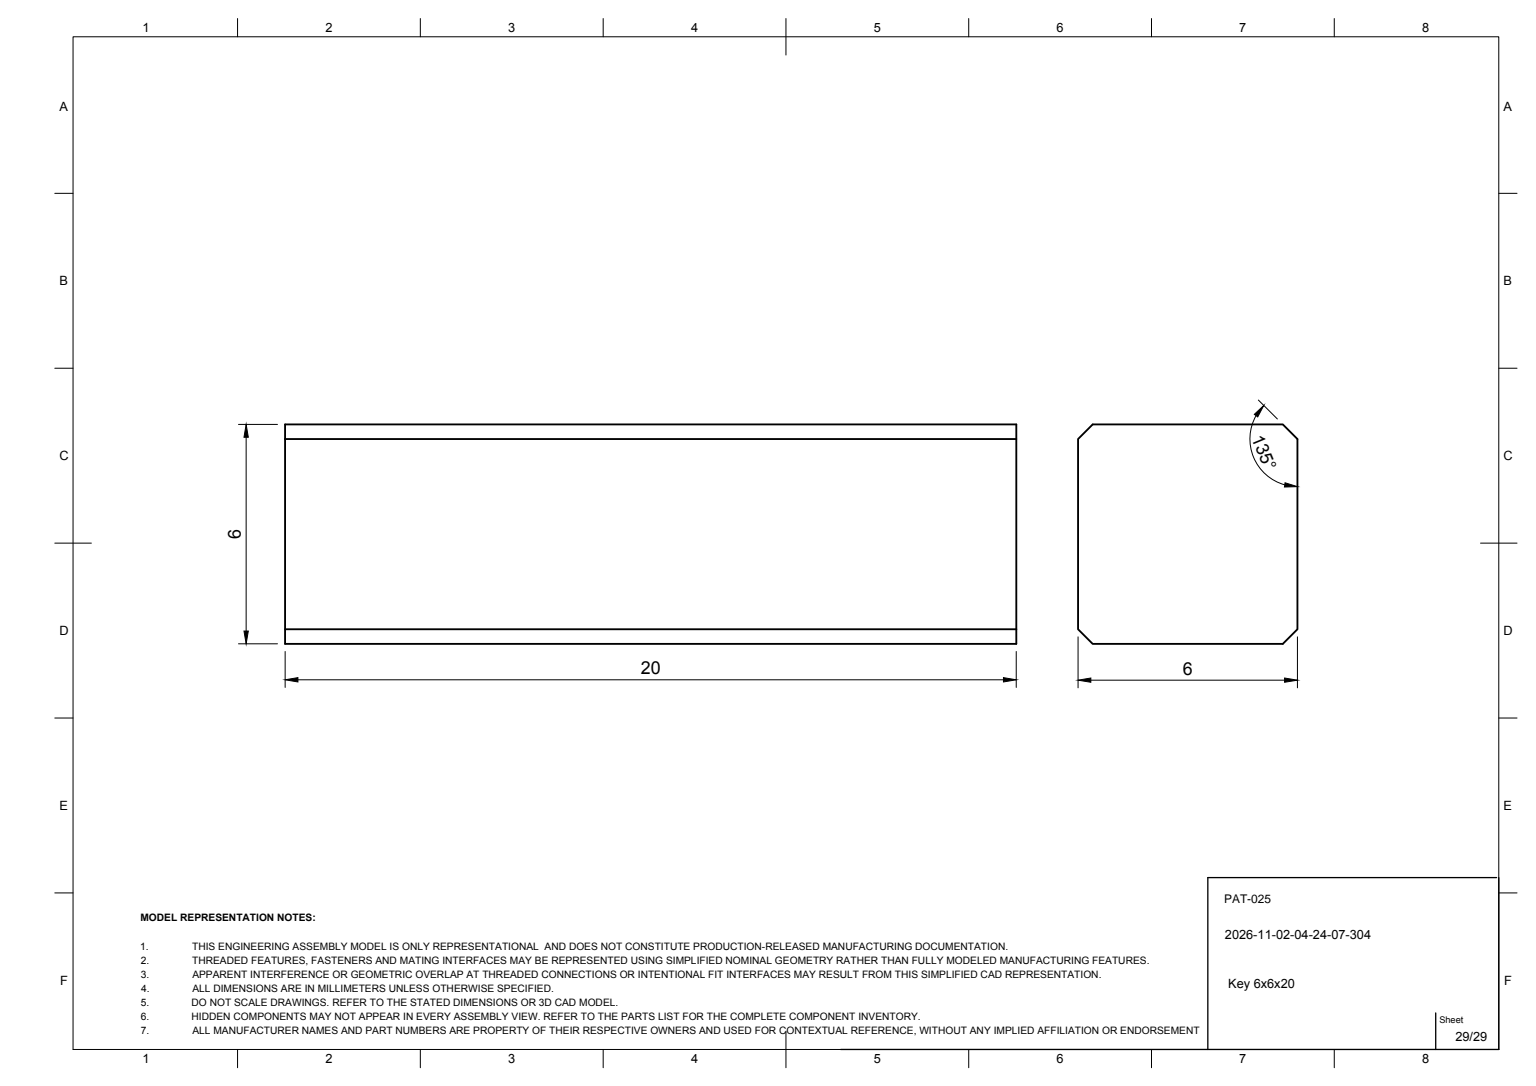
ISO-10303-21;
HEADER;
/* Generated by software containing ST-Developer
 * from STEP Tools, Inc. (www.steptools.com) 
 */

FILE_DESCRIPTION(
/* description */ ('Counter shaft with two pulleys and keyed hub'),
/* implementation_level */ '2;1');

FILE_NAME(
/* name */ 'Key 6x6x20.step',
/* time_stamp */ '2026-10-27T10:46:10-07:00',
/* author */ (''),
/* organization */ (''),
/* preprocessor_version */ 'ST-DEVELOPER v20.2',
/* originating_system */ 'Autodesk Translation Framework v15.17.0.0',
/* authorisation */ '');

FILE_SCHEMA (('AUTOMOTIVE_DESIGN { 1 0 10303 214 3 1 1 }'));
ENDSEC;

DATA;
#10=MECHANICAL_DESIGN_GEOMETRIC_PRESENTATION_REPRESENTATION('',(#314),#10821);
#263=SHAPE_REPRESENTATION_RELATIONSHIP('SRR','None',#10951,#288);
#288=ADVANCED_BREP_SHAPE_REPRESENTATION('',(#338),#10819);
#314=STYLED_ITEM('',(#11135),#338);
#338=MANIFOLD_SOLID_BREP('Body1',#5599);
#569=PLANE('',#6511);
#570=PLANE('',#6512);
#571=PLANE('',#6513);
#572=PLANE('',#6514);
#573=PLANE('',#6515);
#574=PLANE('',#6516);
#575=PLANE('',#6517);
#576=PLANE('',#6518);
#577=PLANE('',#6519);
#578=PLANE('',#6520);
#880=FACE_OUTER_BOUND('',#1284,.T.);
#881=FACE_OUTER_BOUND('',#1285,.T.);
#882=FACE_OUTER_BOUND('',#1286,.T.);
#883=FACE_OUTER_BOUND('',#1287,.T.);
#884=FACE_OUTER_BOUND('',#1288,.T.);
#885=FACE_OUTER_BOUND('',#1289,.T.);
#886=FACE_OUTER_BOUND('',#1290,.T.);
#887=FACE_OUTER_BOUND('',#1291,.T.);
#888=FACE_OUTER_BOUND('',#1292,.T.);
#889=FACE_OUTER_BOUND('',#1293,.T.);
#1284=EDGE_LOOP('',(#5015,#5016,#5017,#5018,#5019,#5020,#5021,#5022));
#1285=EDGE_LOOP('',(#5023,#5024,#5025,#5026));
#1286=EDGE_LOOP('',(#5027,#5028,#5029,#5030));
#1287=EDGE_LOOP('',(#5031,#5032,#5033,#5034));
#1288=EDGE_LOOP('',(#5035,#5036,#5037,#5038));
#1289=EDGE_LOOP('',(#5039,#5040,#5041,#5042,#5043,#5044,#5045,#5046));
#1290=EDGE_LOOP('',(#5047,#5048,#5049,#5050));
#1291=EDGE_LOOP('',(#5051,#5052,#5053,#5054));
#1292=EDGE_LOOP('',(#5055,#5056,#5057,#5058));
#1293=EDGE_LOOP('',(#5059,#5060,#5061,#5062));
#1651=LINE('',#10640,#2040);
#1652=LINE('',#10642,#2041);
#1653=LINE('',#10644,#2042);
#1654=LINE('',#10646,#2043);
#1655=LINE('',#10648,#2044);
#1656=LINE('',#10650,#2045);
#1657=LINE('',#10652,#2046);
#1658=LINE('',#10653,#2047);
#1659=LINE('',#10656,#2048);
#1660=LINE('',#10658,#2049);
#1661=LINE('',#10659,#2050);
#1662=LINE('',#10662,#2051);
#1663=LINE('',#10663,#2052);
#1664=LINE('',#10666,#2053);
#1665=LINE('',#10667,#2054);
#1666=LINE('',#10670,#2055);
#1667=LINE('',#10671,#2056);
#1668=LINE('',#10675,#2057);
#1669=LINE('',#10676,#2058);
#1670=LINE('',#10678,#2059);
#1671=LINE('',#10679,#2060);
#1672=LINE('',#10681,#2061);
#1673=LINE('',#10683,#2062);
#1674=LINE('',#10685,#2063);
#2040=VECTOR('',#8173,1.);
#2041=VECTOR('',#8174,1.);
#2042=VECTOR('',#8175,1.);
#2043=VECTOR('',#8176,1.);
#2044=VECTOR('',#8177,1.);
#2045=VECTOR('',#8178,1.);
#2046=VECTOR('',#8179,1.);
#2047=VECTOR('',#8180,1.);
#2048=VECTOR('',#8183,1.);
#2049=VECTOR('',#8184,1.);
#2050=VECTOR('',#8185,1.);
#2051=VECTOR('',#8188,1.);
#2052=VECTOR('',#8189,1.);
#2053=VECTOR('',#8192,1.);
#2054=VECTOR('',#8193,1.);
#2055=VECTOR('',#8196,1.);
#2056=VECTOR('',#8197,1.);
#2057=VECTOR('',#8200,1.);
#2058=VECTOR('',#8201,1.);
#2059=VECTOR('',#8202,1.);
#2060=VECTOR('',#8203,1.);
#2061=VECTOR('',#8206,1.);
#2062=VECTOR('',#8209,1.);
#2063=VECTOR('',#8212,1.);
#2855=VERTEX_POINT('',#10638);
#2856=VERTEX_POINT('',#10639);
#2857=VERTEX_POINT('',#10641);
#2858=VERTEX_POINT('',#10643);
#2859=VERTEX_POINT('',#10645);
#2860=VERTEX_POINT('',#10647);
#2861=VERTEX_POINT('',#10649);
#2862=VERTEX_POINT('',#10651);
#2863=VERTEX_POINT('',#10655);
#2864=VERTEX_POINT('',#10657);
#2865=VERTEX_POINT('',#10661);
#2866=VERTEX_POINT('',#10665);
#2867=VERTEX_POINT('',#10669);
#2868=VERTEX_POINT('',#10673);
#2869=VERTEX_POINT('',#10674);
#2870=VERTEX_POINT('',#10677);
#3580=EDGE_CURVE('',#2855,#2856,#1651,.T.);
#3581=EDGE_CURVE('',#2857,#2855,#1652,.T.);
#3582=EDGE_CURVE('',#2858,#2857,#1653,.T.);
#3583=EDGE_CURVE('',#2859,#2858,#1654,.T.);
#3584=EDGE_CURVE('',#2860,#2859,#1655,.T.);
#3585=EDGE_CURVE('',#2861,#2860,#1656,.T.);
#3586=EDGE_CURVE('',#2862,#2861,#1657,.T.);
#3587=EDGE_CURVE('',#2856,#2862,#1658,.T.);
#3588=EDGE_CURVE('',#2859,#2863,#1659,.T.);
#3589=EDGE_CURVE('',#2863,#2864,#1660,.T.);
#3590=EDGE_CURVE('',#2864,#2860,#1661,.T.);
#3591=EDGE_CURVE('',#2865,#2858,#1662,.T.);
#3592=EDGE_CURVE('',#2865,#2863,#1663,.T.);
#3593=EDGE_CURVE('',#2857,#2866,#1664,.T.);
#3594=EDGE_CURVE('',#2866,#2865,#1665,.T.);
#3595=EDGE_CURVE('',#2867,#2855,#1666,.T.);
#3596=EDGE_CURVE('',#2867,#2866,#1667,.T.);
#3597=EDGE_CURVE('',#2868,#2869,#1668,.T.);
#3598=EDGE_CURVE('',#2864,#2868,#1669,.T.);
#3599=EDGE_CURVE('',#2870,#2867,#1670,.T.);
#3600=EDGE_CURVE('',#2869,#2870,#1671,.T.);
#3601=EDGE_CURVE('',#2861,#2868,#1672,.T.);
#3602=EDGE_CURVE('',#2856,#2870,#1673,.T.);
#3603=EDGE_CURVE('',#2869,#2862,#1674,.T.);
#5015=ORIENTED_EDGE('',*,*,#3580,.F.);
#5016=ORIENTED_EDGE('',*,*,#3581,.F.);
#5017=ORIENTED_EDGE('',*,*,#3582,.F.);
#5018=ORIENTED_EDGE('',*,*,#3583,.F.);
#5019=ORIENTED_EDGE('',*,*,#3584,.F.);
#5020=ORIENTED_EDGE('',*,*,#3585,.F.);
#5021=ORIENTED_EDGE('',*,*,#3586,.F.);
#5022=ORIENTED_EDGE('',*,*,#3587,.F.);
#5023=ORIENTED_EDGE('',*,*,#3584,.T.);
#5024=ORIENTED_EDGE('',*,*,#3588,.T.);
#5025=ORIENTED_EDGE('',*,*,#3589,.T.);
#5026=ORIENTED_EDGE('',*,*,#3590,.T.);
#5027=ORIENTED_EDGE('',*,*,#3583,.T.);
#5028=ORIENTED_EDGE('',*,*,#3591,.F.);
#5029=ORIENTED_EDGE('',*,*,#3592,.T.);
#5030=ORIENTED_EDGE('',*,*,#3588,.F.);
#5031=ORIENTED_EDGE('',*,*,#3582,.T.);
#5032=ORIENTED_EDGE('',*,*,#3593,.T.);
#5033=ORIENTED_EDGE('',*,*,#3594,.T.);
#5034=ORIENTED_EDGE('',*,*,#3591,.T.);
#5035=ORIENTED_EDGE('',*,*,#3581,.T.);
#5036=ORIENTED_EDGE('',*,*,#3595,.F.);
#5037=ORIENTED_EDGE('',*,*,#3596,.T.);
#5038=ORIENTED_EDGE('',*,*,#3593,.F.);
#5039=ORIENTED_EDGE('',*,*,#3597,.F.);
#5040=ORIENTED_EDGE('',*,*,#3598,.F.);
#5041=ORIENTED_EDGE('',*,*,#3589,.F.);
#5042=ORIENTED_EDGE('',*,*,#3592,.F.);
#5043=ORIENTED_EDGE('',*,*,#3594,.F.);
#5044=ORIENTED_EDGE('',*,*,#3596,.F.);
#5045=ORIENTED_EDGE('',*,*,#3599,.F.);
#5046=ORIENTED_EDGE('',*,*,#3600,.F.);
#5047=ORIENTED_EDGE('',*,*,#3585,.T.);
#5048=ORIENTED_EDGE('',*,*,#3590,.F.);
#5049=ORIENTED_EDGE('',*,*,#3598,.T.);
#5050=ORIENTED_EDGE('',*,*,#3601,.F.);
#5051=ORIENTED_EDGE('',*,*,#3580,.T.);
#5052=ORIENTED_EDGE('',*,*,#3602,.T.);
#5053=ORIENTED_EDGE('',*,*,#3599,.T.);
#5054=ORIENTED_EDGE('',*,*,#3595,.T.);
#5055=ORIENTED_EDGE('',*,*,#3586,.T.);
#5056=ORIENTED_EDGE('',*,*,#3601,.T.);
#5057=ORIENTED_EDGE('',*,*,#3597,.T.);
#5058=ORIENTED_EDGE('',*,*,#3603,.T.);
#5059=ORIENTED_EDGE('',*,*,#3587,.T.);
#5060=ORIENTED_EDGE('',*,*,#3603,.F.);
#5061=ORIENTED_EDGE('',*,*,#3600,.T.);
#5062=ORIENTED_EDGE('',*,*,#3602,.F.);
#5551=ADVANCED_FACE('',(#880),#569,.F.);
#5552=ADVANCED_FACE('',(#881),#570,.T.);
#5553=ADVANCED_FACE('',(#882),#571,.T.);
#5554=ADVANCED_FACE('',(#883),#572,.T.);
#5555=ADVANCED_FACE('',(#884),#573,.T.);
#5556=ADVANCED_FACE('',(#885),#574,.T.);
#5557=ADVANCED_FACE('',(#886),#575,.F.);
#5558=ADVANCED_FACE('',(#887),#576,.T.);
#5559=ADVANCED_FACE('',(#888),#577,.T.);
#5560=ADVANCED_FACE('',(#889),#578,.T.);
#5599=CLOSED_SHELL('',(#5551,#5552,#5553,#5554,#5555,#5556,#5557,#5558,
#5559,#5560));
#6510=AXIS2_PLACEMENT_3D('',#10636,#8169,#8170);
#6511=AXIS2_PLACEMENT_3D('',#10637,#8171,#8172);
#6512=AXIS2_PLACEMENT_3D('',#10654,#8181,#8182);
#6513=AXIS2_PLACEMENT_3D('',#10660,#8186,#8187);
#6514=AXIS2_PLACEMENT_3D('',#10664,#8190,#8191);
#6515=AXIS2_PLACEMENT_3D('',#10668,#8194,#8195);
#6516=AXIS2_PLACEMENT_3D('',#10672,#8198,#8199);
#6517=AXIS2_PLACEMENT_3D('',#10680,#8204,#8205);
#6518=AXIS2_PLACEMENT_3D('',#10682,#8207,#8208);
#6519=AXIS2_PLACEMENT_3D('',#10684,#8210,#8211);
#6520=AXIS2_PLACEMENT_3D('',#10686,#8213,#8214);
#8169=DIRECTION('axis',(0.,0.,1.));
#8170=DIRECTION('refdir',(1.,0.,0.));
#8171=DIRECTION('center_axis',(1.,0.,0.));
#8172=DIRECTION('ref_axis',(0.,0.,-1.));
#8173=DIRECTION('',(0.,-0.707106781186547,-0.707106781186548));
#8174=DIRECTION('',(0.,-1.,0.));
#8175=DIRECTION('',(0.,-0.707106781186547,0.707106781186548));
#8176=DIRECTION('',(0.,0.,1.));
#8177=DIRECTION('',(0.,0.707106781186547,0.707106781186548));
#8178=DIRECTION('',(0.,1.,0.));
#8179=DIRECTION('',(0.,0.707106781186547,-0.707106781186548));
#8180=DIRECTION('',(0.,0.,-1.));
#8181=DIRECTION('center_axis',(0.,0.707106781186548,-0.707106781186547));
#8182=DIRECTION('ref_axis',(-1.,0.,0.));
#8183=DIRECTION('',(1.,0.,0.));
#8184=DIRECTION('',(0.,-0.707106781186547,-0.707106781186548));
#8185=DIRECTION('',(-1.,0.,0.));
#8186=DIRECTION('center_axis',(0.,1.,0.));
#8187=DIRECTION('ref_axis',(-1.,0.,0.));
#8188=DIRECTION('',(-1.,0.,0.));
#8189=DIRECTION('',(0.,0.,-1.));
#8190=DIRECTION('center_axis',(0.,0.707106781186548,0.707106781186547));
#8191=DIRECTION('ref_axis',(1.,0.,0.));
#8192=DIRECTION('',(1.,0.,0.));
#8193=DIRECTION('',(0.,0.707106781186547,-0.707106781186548));
#8194=DIRECTION('center_axis',(0.,0.,1.));
#8195=DIRECTION('ref_axis',(1.,0.,0.));
#8196=DIRECTION('',(-1.,0.,0.));
#8197=DIRECTION('',(0.,1.,0.));
#8198=DIRECTION('center_axis',(1.,0.,0.));
#8199=DIRECTION('ref_axis',(0.,0.,-1.));
#8200=DIRECTION('',(0.,-0.707106781186547,0.707106781186548));
#8201=DIRECTION('',(0.,-1.,0.));
#8202=DIRECTION('',(0.,0.707106781186547,0.707106781186548));
#8203=DIRECTION('',(0.,0.,1.));
#8204=DIRECTION('center_axis',(0.,0.,1.));
#8205=DIRECTION('ref_axis',(1.,0.,0.));
#8206=DIRECTION('',(1.,0.,0.));
#8207=DIRECTION('center_axis',(0.,-0.707106781186548,0.707106781186547));
#8208=DIRECTION('ref_axis',(1.,0.,0.));
#8209=DIRECTION('',(1.,0.,0.));
#8210=DIRECTION('center_axis',(0.,-0.707106781186548,-0.707106781186547));
#8211=DIRECTION('ref_axis',(-1.,0.,0.));
#8212=DIRECTION('',(-1.,0.,0.));
#8213=DIRECTION('center_axis',(0.,-1.,0.));
#8214=DIRECTION('ref_axis',(1.,0.,0.));
#10636=CARTESIAN_POINT('',(0.,0.,0.));
#10637=CARTESIAN_POINT('Origin',(-1.,0.,0.35));
#10638=CARTESIAN_POINT('',(-1.,-0.26,0.6));
#10639=CARTESIAN_POINT('',(-1.,-0.3,0.56));
#10640=CARTESIAN_POINT('',(-1.,-0.2675,0.5925));
#10641=CARTESIAN_POINT('',(-1.,0.26,0.6));
#10642=CARTESIAN_POINT('',(-1.,0.,0.6));
#10643=CARTESIAN_POINT('',(-1.,0.3,0.56));
#10644=CARTESIAN_POINT('',(-1.,0.2675,0.5925));
#10645=CARTESIAN_POINT('',(-1.,0.3,0.04));
#10646=CARTESIAN_POINT('',(-1.,0.3,0.175));
#10647=CARTESIAN_POINT('',(-1.,0.26,0.));
#10648=CARTESIAN_POINT('',(-1.,0.2925,0.0325));
#10649=CARTESIAN_POINT('',(-1.,-0.26,0.));
#10650=CARTESIAN_POINT('',(-1.,0.,0.));
#10651=CARTESIAN_POINT('',(-1.,-0.3,0.04));
#10652=CARTESIAN_POINT('',(-1.,-0.2925,0.0325));
#10653=CARTESIAN_POINT('',(-1.,-0.3,0.175));
#10654=CARTESIAN_POINT('Origin',(0.75,0.28,0.02));
#10655=CARTESIAN_POINT('',(1.,0.3,0.04));
#10656=CARTESIAN_POINT('',(0.75,0.3,0.04));
#10657=CARTESIAN_POINT('',(1.,0.26,0.));
#10658=CARTESIAN_POINT('',(1.,0.2925,0.0325));
#10659=CARTESIAN_POINT('',(0.75,0.26,0.));
#10660=CARTESIAN_POINT('Origin',(1.5,0.3,0.));
#10661=CARTESIAN_POINT('',(1.,0.3,0.56));
#10662=CARTESIAN_POINT('',(0.75,0.3,0.56));
#10663=CARTESIAN_POINT('',(1.,0.3,0.175));
#10664=CARTESIAN_POINT('Origin',(0.75,0.28,0.58));
#10665=CARTESIAN_POINT('',(1.,0.26,0.6));
#10666=CARTESIAN_POINT('',(0.75,0.26,0.6));
#10667=CARTESIAN_POINT('',(1.,0.2675,0.5925));
#10668=CARTESIAN_POINT('Origin',(0.,0.,0.6));
#10669=CARTESIAN_POINT('',(1.,-0.26,0.6));
#10670=CARTESIAN_POINT('',(-0.75,-0.26,0.6));
#10671=CARTESIAN_POINT('',(1.,0.,0.6));
#10672=CARTESIAN_POINT('Origin',(1.,0.,0.35));
#10673=CARTESIAN_POINT('',(1.,-0.26,0.));
#10674=CARTESIAN_POINT('',(1.,-0.3,0.04));
#10675=CARTESIAN_POINT('',(1.,-0.2925,0.0325));
#10676=CARTESIAN_POINT('',(1.,0.,0.));
#10677=CARTESIAN_POINT('',(1.,-0.3,0.56));
#10678=CARTESIAN_POINT('',(1.,-0.2675,0.5925));
#10679=CARTESIAN_POINT('',(1.,-0.3,0.175));
#10680=CARTESIAN_POINT('Origin',(0.,0.,0.));
#10681=CARTESIAN_POINT('',(-0.75,-0.26,0.));
#10682=CARTESIAN_POINT('Origin',(-0.75,-0.28,0.58));
#10683=CARTESIAN_POINT('',(-0.75,-0.3,0.56));
#10684=CARTESIAN_POINT('Origin',(-0.75,-0.28,0.02));
#10685=CARTESIAN_POINT('',(-0.75,-0.3,0.04));
#10686=CARTESIAN_POINT('Origin',(-1.5,-0.3,0.));
#10789=UNCERTAINTY_MEASURE_WITH_UNIT(LENGTH_MEASURE(0.001),#10822,
'DISTANCE_ACCURACY_VALUE',
'Maximum model space distance between geometric entities at asserted c
onnectivities');
#10791=UNCERTAINTY_MEASURE_WITH_UNIT(LENGTH_MEASURE(0.001),#10822,
'DISTANCE_ACCURACY_VALUE',
'Maximum model space distance between geometric entities at asserted c
onnectivities');
#10819=(
GEOMETRIC_REPRESENTATION_CONTEXT(3)
GLOBAL_UNCERTAINTY_ASSIGNED_CONTEXT((#10789))
GLOBAL_UNIT_ASSIGNED_CONTEXT((#10822,#10824,#10825))
REPRESENTATION_CONTEXT('','3D')
);
#10821=(
GEOMETRIC_REPRESENTATION_CONTEXT(3)
GLOBAL_UNCERTAINTY_ASSIGNED_CONTEXT((#10791))
GLOBAL_UNIT_ASSIGNED_CONTEXT((#10822,#10824,#10825))
REPRESENTATION_CONTEXT('','3D')
);
#10822=(
LENGTH_UNIT()
NAMED_UNIT(*)
SI_UNIT(.CENTI.,.METRE.)
);
#10824=(
NAMED_UNIT(*)
PLANE_ANGLE_UNIT()
SI_UNIT($,.RADIAN.)
);
#10825=(
NAMED_UNIT(*)
SI_UNIT($,.STERADIAN.)
SOLID_ANGLE_UNIT()
);
#10853=SHAPE_DEFINITION_REPRESENTATION(#10901,#10951);
#10901=PRODUCT_DEFINITION_SHAPE('',$,#10981);
#10951=SHAPE_REPRESENTATION('',(#6510),#10819);
#10953=PRODUCT_DEFINITION_CONTEXT('part definition',#11042,'design');
#10981=PRODUCT_DEFINITION('Key 6x6x20','Key 6x6x20',#11010,#10953);
#11010=PRODUCT_DEFINITION_FORMATION('',$,#11071);
#11042=APPLICATION_CONTEXT(
'Core Data for Automotive Mechanical Design Process');
#11043=PRODUCT_CONTEXT('part definition',#11042,'mechanical');
#11071=PRODUCT('Key 6x6x20','Key 6x6x20','Key 6x6x20',(#11043));
#11129=COLOUR_RGB('Grey',0.48,0.52,0.57);
#11130=FILL_AREA_STYLE_COLOUR('',#11129);
#11131=FILL_AREA_STYLE('',(#11130));
#11132=SURFACE_STYLE_FILL_AREA(#11131);
#11133=SURFACE_SIDE_STYLE('',(#11132));
#11134=SURFACE_STYLE_USAGE(.BOTH.,#11133);
#11135=PRESENTATION_STYLE_ASSIGNMENT((#11134));
ENDSEC;
END-ISO-10303-21;
